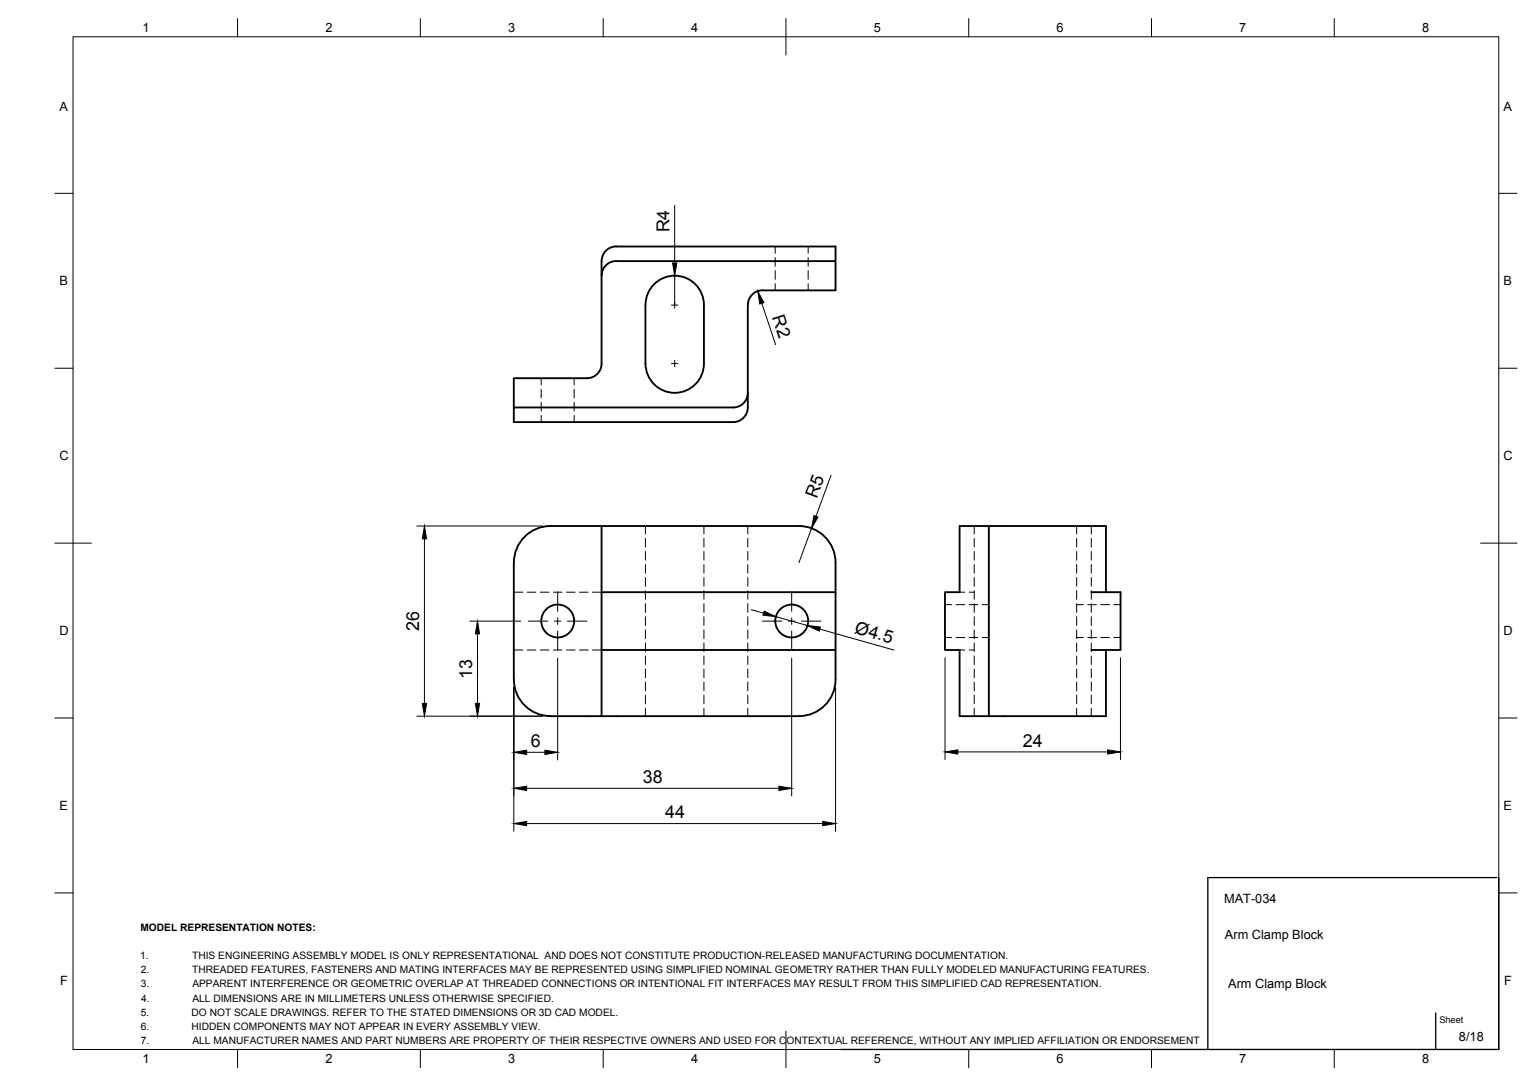
ISO-10303-21;
HEADER;
/* Generated by software containing ST-Developer
 * from STEP Tools, Inc. (www.steptools.com) 
 */

FILE_DESCRIPTION(
/* description */ ('STEP AP214'),
/* implementation_level */ '2;1');

FILE_NAME(
/* name */ 'Arm Clamp Block.step',
/* time_stamp */ '2026-11-14T09:24:36-08:00',
/* author */ (''),
/* organization */ (''),
/* preprocessor_version */ 'ST-DEVELOPER v20.2',
/* originating_system */ 'Autodesk Translation Framework v15.17.0.0',
/* authorisation */ '');

FILE_SCHEMA (('AUTOMOTIVE_DESIGN { 1 0 10303 214 3 1 1 }'));
ENDSEC;

DATA;
#10=MECHANICAL_DESIGN_GEOMETRIC_PRESENTATION_REPRESENTATION('',(#214),#18867);
#182=SHAPE_REPRESENTATION_RELATIONSHIP('SRR','None',#18946,#198);
#198=ADVANCED_BREP_SHAPE_REPRESENTATION('',(#238),#18862);
#214=STYLED_ITEM('',(#19026),#238);
#238=MANIFOLD_SOLID_BREP('Body1',#10969);
#356=FACE_BOUND('',#1900,.T.);
#357=FACE_BOUND('',#1905,.T.);
#358=FACE_BOUND('',#1908,.T.);
#359=FACE_BOUND('',#1910,.T.);
#360=FACE_BOUND('',#1924,.T.);
#361=FACE_BOUND('',#1928,.T.);
#666=PLANE('',#12022);
#667=PLANE('',#12024);
#668=PLANE('',#12026);
#669=PLANE('',#12028);
#670=PLANE('',#12029);
#671=PLANE('',#12032);
#672=PLANE('',#12033);
#673=PLANE('',#12035);
#674=PLANE('',#12036);
#675=PLANE('',#12039);
#676=PLANE('',#12040);
#677=PLANE('',#12047);
#678=PLANE('',#12055);
#679=PLANE('',#12057);
#680=PLANE('',#12064);
#681=PLANE('',#12067);
#682=PLANE('',#12070);
#683=PLANE('',#12071);
#684=PLANE('',#12074);
#685=PLANE('',#12077);
#1192=FACE_OUTER_BOUND('',#1893,.T.);
#1193=FACE_OUTER_BOUND('',#1894,.T.);
#1194=FACE_OUTER_BOUND('',#1895,.T.);
#1195=FACE_OUTER_BOUND('',#1896,.T.);
#1196=FACE_OUTER_BOUND('',#1897,.T.);
#1197=FACE_OUTER_BOUND('',#1898,.T.);
#1198=FACE_OUTER_BOUND('',#1899,.T.);
#1199=FACE_OUTER_BOUND('',#1901,.T.);
#1200=FACE_OUTER_BOUND('',#1902,.T.);
#1201=FACE_OUTER_BOUND('',#1903,.T.);
#1202=FACE_OUTER_BOUND('',#1904,.T.);
#1203=FACE_OUTER_BOUND('',#1906,.T.);
#1204=FACE_OUTER_BOUND('',#1907,.T.);
#1205=FACE_OUTER_BOUND('',#1909,.T.);
#1206=FACE_OUTER_BOUND('',#1911,.T.);
#1207=FACE_OUTER_BOUND('',#1912,.T.);
#1208=FACE_OUTER_BOUND('',#1913,.T.);
#1209=FACE_OUTER_BOUND('',#1914,.T.);
#1210=FACE_OUTER_BOUND('',#1915,.T.);
#1211=FACE_OUTER_BOUND('',#1916,.T.);
#1212=FACE_OUTER_BOUND('',#1917,.T.);
#1213=FACE_OUTER_BOUND('',#1918,.T.);
#1214=FACE_OUTER_BOUND('',#1919,.T.);
#1215=FACE_OUTER_BOUND('',#1920,.T.);
#1216=FACE_OUTER_BOUND('',#1921,.T.);
#1217=FACE_OUTER_BOUND('',#1922,.T.);
#1218=FACE_OUTER_BOUND('',#1923,.T.);
#1219=FACE_OUTER_BOUND('',#1925,.T.);
#1220=FACE_OUTER_BOUND('',#1926,.T.);
#1221=FACE_OUTER_BOUND('',#1927,.T.);
#1222=FACE_OUTER_BOUND('',#1929,.T.);
#1223=FACE_OUTER_BOUND('',#1930,.T.);
#1224=FACE_OUTER_BOUND('',#1931,.T.);
#1225=FACE_OUTER_BOUND('',#1932,.T.);
#1226=FACE_OUTER_BOUND('',#1933,.T.);
#1227=FACE_OUTER_BOUND('',#1934,.T.);
#1893=EDGE_LOOP('',(#9564,#9565,#9566,#9567));
#1894=EDGE_LOOP('',(#9568,#9569,#9570,#9571));
#1895=EDGE_LOOP('',(#9572,#9573,#9574,#9575,#9576));
#1896=EDGE_LOOP('',(#9577,#9578,#9579,#9580,#9581));
#1897=EDGE_LOOP('',(#9582,#9583,#9584,#9585,#9586));
#1898=EDGE_LOOP('',(#9587,#9588,#9589,#9590,#9591,#9592,#9593,#9594));
#1899=EDGE_LOOP('',(#9595,#9596,#9597,#9598,#9599,#9600));
#1900=EDGE_LOOP('',(#9601));
#1901=EDGE_LOOP('',(#9602,#9603,#9604,#9605,#9606,#9607,#9608,#9609));
#1902=EDGE_LOOP('',(#9610,#9611,#9612,#9613,#9614));
#1903=EDGE_LOOP('',(#9615,#9616,#9617,#9618,#9619,#9620,#9621,#9622));
#1904=EDGE_LOOP('',(#9623,#9624,#9625,#9626,#9627,#9628));
#1905=EDGE_LOOP('',(#9629));
#1906=EDGE_LOOP('',(#9630,#9631,#9632,#9633,#9634,#9635,#9636,#9637));
#1907=EDGE_LOOP('',(#9638,#9639,#9640,#9641,#9642,#9643,#9644,#9645,#9646,
#9647,#9648,#9649));
#1908=EDGE_LOOP('',(#9650,#9651,#9652,#9653));
#1909=EDGE_LOOP('',(#9654,#9655,#9656,#9657,#9658,#9659,#9660,#9661,#9662,
#9663,#9664,#9665));
#1910=EDGE_LOOP('',(#9666,#9667,#9668,#9669));
#1911=EDGE_LOOP('',(#9670,#9671,#9672,#9673));
#1912=EDGE_LOOP('',(#9674,#9675,#9676,#9677));
#1913=EDGE_LOOP('',(#9678,#9679,#9680,#9681));
#1914=EDGE_LOOP('',(#9682,#9683,#9684,#9685));
#1915=EDGE_LOOP('',(#9686,#9687,#9688,#9689));
#1916=EDGE_LOOP('',(#9690,#9691,#9692,#9693));
#1917=EDGE_LOOP('',(#9694,#9695,#9696,#9697));
#1918=EDGE_LOOP('',(#9698,#9699,#9700,#9701));
#1919=EDGE_LOOP('',(#9702,#9703,#9704,#9705));
#1920=EDGE_LOOP('',(#9706,#9707,#9708,#9709));
#1921=EDGE_LOOP('',(#9710,#9711,#9712,#9713,#9714,#9715));
#1922=EDGE_LOOP('',(#9716,#9717,#9718,#9719,#9720,#9721));
#1923=EDGE_LOOP('',(#9722,#9723,#9724,#9725));
#1924=EDGE_LOOP('',(#9726));
#1925=EDGE_LOOP('',(#9727,#9728,#9729,#9730,#9731,#9732));
#1926=EDGE_LOOP('',(#9733,#9734,#9735,#9736,#9737,#9738));
#1927=EDGE_LOOP('',(#9739,#9740,#9741,#9742));
#1928=EDGE_LOOP('',(#9743));
#1929=EDGE_LOOP('',(#9744,#9745,#9746,#9747));
#1930=EDGE_LOOP('',(#9748,#9749,#9750,#9751));
#1931=EDGE_LOOP('',(#9752,#9753,#9754,#9755));
#1932=EDGE_LOOP('',(#9756,#9757,#9758,#9759));
#1933=EDGE_LOOP('',(#9760,#9761,#9762,#9763));
#1934=EDGE_LOOP('',(#9764,#9765,#9766,#9767));
#2894=LINE('',#18183,#3908);
#2895=LINE('',#18189,#3909);
#2896=LINE('',#18194,#3910);
#2897=LINE('',#18196,#3911);
#2898=LINE('',#18198,#3912);
#2899=LINE('',#18200,#3913);
#2900=LINE('',#18205,#3914);
#2901=LINE('',#18207,#3915);
#2902=LINE('',#18209,#3916);
#2903=LINE('',#18211,#3917);
#2904=LINE('',#18216,#3918);
#2905=LINE('',#18218,#3919);
#2906=LINE('',#18220,#3920);
#2907=LINE('',#18223,#3921);
#2908=LINE('',#18226,#3922);
#2909=LINE('',#18228,#3923);
#2910=LINE('',#18229,#3924);
#2911=LINE('',#18231,#3925);
#2912=LINE('',#18233,#3926);
#2913=LINE('',#18234,#3927);
#2914=LINE('',#18239,#3928);
#2915=LINE('',#18241,#3929);
#2916=LINE('',#18243,#3930);
#2917=LINE('',#18248,#3931);
#2918=LINE('',#18250,#3932);
#2919=LINE('',#18252,#3933);
#2920=LINE('',#18254,#3934);
#2921=LINE('',#18256,#3935);
#2922=LINE('',#18258,#3936);
#2923=LINE('',#18260,#3937);
#2924=LINE('',#18261,#3938);
#2925=LINE('',#18265,#3939);
#2926=LINE('',#18267,#3940);
#2927=LINE('',#18269,#3941);
#2928=LINE('',#18272,#3942);
#2929=LINE('',#18276,#3943);
#2930=LINE('',#18277,#3944);
#2931=LINE('',#18279,#3945);
#2932=LINE('',#18281,#3946);
#2933=LINE('',#18282,#3947);
#2934=LINE('',#18283,#3948);
#2935=LINE('',#18287,#3949);
#2936=LINE('',#18292,#3950);
#2937=LINE('',#18293,#3951);
#2938=LINE('',#18297,#3952);
#2939=LINE('',#18299,#3953);
#2940=LINE('',#18301,#3954);
#2941=LINE('',#18303,#3955);
#2942=LINE('',#18305,#3956);
#2943=LINE('',#18307,#3957);
#2944=LINE('',#18309,#3958);
#2945=LINE('',#18310,#3959);
#2946=LINE('',#18313,#3960);
#2947=LINE('',#18316,#3961);
#2948=LINE('',#18322,#3962);
#2949=LINE('',#18325,#3963);
#2950=LINE('',#18329,#3964);
#2951=LINE('',#18332,#3965);
#2952=LINE('',#18335,#3966);
#2953=LINE('',#18339,#3967);
#2954=LINE('',#18342,#3968);
#2955=LINE('',#18343,#3969);
#2956=LINE('',#18345,#3970);
#2957=LINE('',#18347,#3971);
#2958=LINE('',#18359,#3972);
#2959=LINE('',#18362,#3973);
#2960=LINE('',#18366,#3974);
#2961=LINE('',#18371,#3975);
#2962=LINE('',#18374,#3976);
#2963=LINE('',#18378,#3977);
#3908=VECTOR('',#14868,2.25);
#3909=VECTOR('',#14875,2.25);
#3910=VECTOR('',#14880,1000.);
#3911=VECTOR('',#14881,1000.);
#3912=VECTOR('',#14882,1000.);
#3913=VECTOR('',#14883,1000.);
#3914=VECTOR('',#14888,1000.);
#3915=VECTOR('',#14889,1000.);
#3916=VECTOR('',#14890,1000.);
#3917=VECTOR('',#14891,1000.);
#3918=VECTOR('',#14896,1000.);
#3919=VECTOR('',#14897,1000.);
#3920=VECTOR('',#14898,1000.);
#3921=VECTOR('',#14901,1000.);
#3922=VECTOR('',#14904,1000.);
#3923=VECTOR('',#14905,1000.);
#3924=VECTOR('',#14906,1000.);
#3925=VECTOR('',#14907,1000.);
#3926=VECTOR('',#14908,1000.);
#3927=VECTOR('',#14909,1000.);
#3928=VECTOR('',#14914,1000.);
#3929=VECTOR('',#14915,1000.);
#3930=VECTOR('',#14916,1000.);
#3931=VECTOR('',#14921,1000.);
#3932=VECTOR('',#14922,1000.);
#3933=VECTOR('',#14923,1000.);
#3934=VECTOR('',#14924,1000.);
#3935=VECTOR('',#14925,1000.);
#3936=VECTOR('',#14926,1000.);
#3937=VECTOR('',#14927,1000.);
#3938=VECTOR('',#14928,1000.);
#3939=VECTOR('',#14931,1000.);
#3940=VECTOR('',#14932,1000.);
#3941=VECTOR('',#14933,1000.);
#3942=VECTOR('',#14936,1000.);
#3943=VECTOR('',#14939,1000.);
#3944=VECTOR('',#14940,1000.);
#3945=VECTOR('',#14941,1000.);
#3946=VECTOR('',#14942,1000.);
#3947=VECTOR('',#14943,1000.);
#3948=VECTOR('',#14944,1000.);
#3949=VECTOR('',#14947,1000.);
#3950=VECTOR('',#14952,1000.);
#3951=VECTOR('',#14953,1000.);
#3952=VECTOR('',#14956,1000.);
#3953=VECTOR('',#14957,1000.);
#3954=VECTOR('',#14958,1000.);
#3955=VECTOR('',#14959,1000.);
#3956=VECTOR('',#14960,1000.);
#3957=VECTOR('',#14961,1000.);
#3958=VECTOR('',#14962,1000.);
#3959=VECTOR('',#14963,1000.);
#3960=VECTOR('',#14968,1000.);
#3961=VECTOR('',#14973,1000.);
#3962=VECTOR('',#14978,1000.);
#3963=VECTOR('',#14981,1000.);
#3964=VECTOR('',#14988,1000.);
#3965=VECTOR('',#14993,1000.);
#3966=VECTOR('',#14994,1000.);
#3967=VECTOR('',#14997,1000.);
#3968=VECTOR('',#15002,1000.);
#3969=VECTOR('',#15003,1000.);
#3970=VECTOR('',#15006,1000.);
#3971=VECTOR('',#15009,1000.);
#3972=VECTOR('',#15030,1000.);
#3973=VECTOR('',#15033,1000.);
#3974=VECTOR('',#15040,1000.);
#3975=VECTOR('',#15047,1000.);
#3976=VECTOR('',#15050,1000.);
#3977=VECTOR('',#15057,1000.);
#4448=CIRCLE('',#12017,2.25);
#4449=CIRCLE('',#12018,2.25);
#4450=CIRCLE('',#12020,2.25);
#4451=CIRCLE('',#12021,2.25);
#4452=CIRCLE('',#12023,5.);
#4453=CIRCLE('',#12025,5.);
#4454=CIRCLE('',#12027,5.);
#4455=CIRCLE('',#12030,5.);
#4456=CIRCLE('',#12031,5.);
#4457=CIRCLE('',#12034,5.);
#4458=CIRCLE('',#12037,5.);
#4459=CIRCLE('',#12038,5.);
#4460=CIRCLE('',#12041,2.);
#4461=CIRCLE('',#12042,2.);
#4462=CIRCLE('',#12043,2.);
#4463=CIRCLE('',#12044,2.);
#4464=CIRCLE('',#12045,4.);
#4465=CIRCLE('',#12046,4.);
#4466=CIRCLE('',#12048,2.);
#4467=CIRCLE('',#12049,2.);
#4468=CIRCLE('',#12050,2.);
#4469=CIRCLE('',#12051,2.);
#4470=CIRCLE('',#12052,4.);
#4471=CIRCLE('',#12053,4.);
#4472=CIRCLE('',#12065,2.);
#4473=CIRCLE('',#12066,2.);
#4474=CIRCLE('',#12068,2.);
#4475=CIRCLE('',#12069,2.);
#4476=CIRCLE('',#12072,2.);
#4477=CIRCLE('',#12073,2.);
#4478=CIRCLE('',#12075,2.);
#4479=CIRCLE('',#12076,2.);
#5388=VERTEX_POINT('',#18180);
#5389=VERTEX_POINT('',#18182);
#5390=VERTEX_POINT('',#18186);
#5391=VERTEX_POINT('',#18188);
#5392=VERTEX_POINT('',#18192);
#5393=VERTEX_POINT('',#18193);
#5394=VERTEX_POINT('',#18195);
#5395=VERTEX_POINT('',#18197);
#5396=VERTEX_POINT('',#18199);
#5397=VERTEX_POINT('',#18203);
#5398=VERTEX_POINT('',#18204);
#5399=VERTEX_POINT('',#18206);
#5400=VERTEX_POINT('',#18208);
#5401=VERTEX_POINT('',#18210);
#5402=VERTEX_POINT('',#18214);
#5403=VERTEX_POINT('',#18215);
#5404=VERTEX_POINT('',#18217);
#5405=VERTEX_POINT('',#18219);
#5406=VERTEX_POINT('',#18221);
#5407=VERTEX_POINT('',#18225);
#5408=VERTEX_POINT('',#18227);
#5409=VERTEX_POINT('',#18230);
#5410=VERTEX_POINT('',#18232);
#5411=VERTEX_POINT('',#18236);
#5412=VERTEX_POINT('',#18238);
#5413=VERTEX_POINT('',#18240);
#5414=VERTEX_POINT('',#18242);
#5415=VERTEX_POINT('',#18246);
#5416=VERTEX_POINT('',#18247);
#5417=VERTEX_POINT('',#18249);
#5418=VERTEX_POINT('',#18251);
#5419=VERTEX_POINT('',#18253);
#5420=VERTEX_POINT('',#18255);
#5421=VERTEX_POINT('',#18257);
#5422=VERTEX_POINT('',#18259);
#5423=VERTEX_POINT('',#18263);
#5424=VERTEX_POINT('',#18264);
#5425=VERTEX_POINT('',#18266);
#5426=VERTEX_POINT('',#18268);
#5427=VERTEX_POINT('',#18270);
#5428=VERTEX_POINT('',#18274);
#5429=VERTEX_POINT('',#18275);
#5430=VERTEX_POINT('',#18278);
#5431=VERTEX_POINT('',#18280);
#5432=VERTEX_POINT('',#18285);
#5433=VERTEX_POINT('',#18286);
#5434=VERTEX_POINT('',#18289);
#5435=VERTEX_POINT('',#18291);
#5436=VERTEX_POINT('',#18295);
#5437=VERTEX_POINT('',#18296);
#5438=VERTEX_POINT('',#18298);
#5439=VERTEX_POINT('',#18300);
#5440=VERTEX_POINT('',#18302);
#5441=VERTEX_POINT('',#18304);
#5442=VERTEX_POINT('',#18306);
#5443=VERTEX_POINT('',#18308);
#5444=VERTEX_POINT('',#18318);
#5445=VERTEX_POINT('',#18319);
#5446=VERTEX_POINT('',#18321);
#5447=VERTEX_POINT('',#18323);
#5448=VERTEX_POINT('',#18333);
#5449=VERTEX_POINT('',#18334);
#5450=VERTEX_POINT('',#18336);
#5451=VERTEX_POINT('',#18338);
#5452=VERTEX_POINT('',#18357);
#5453=VERTEX_POINT('',#18361);
#5454=VERTEX_POINT('',#18369);
#5455=VERTEX_POINT('',#18373);
#6815=EDGE_CURVE('',#5388,#5388,#4448,.T.);
#6816=EDGE_CURVE('',#5388,#5389,#2894,.T.);
#6817=EDGE_CURVE('',#5389,#5389,#4449,.T.);
#6818=EDGE_CURVE('',#5390,#5390,#4450,.T.);
#6819=EDGE_CURVE('',#5390,#5391,#2895,.T.);
#6820=EDGE_CURVE('',#5391,#5391,#4451,.T.);
#6821=EDGE_CURVE('',#5392,#5393,#2896,.T.);
#6822=EDGE_CURVE('',#5392,#5394,#2897,.T.);
#6823=EDGE_CURVE('',#5395,#5394,#2898,.T.);
#6824=EDGE_CURVE('',#5396,#5395,#2899,.T.);
#6825=EDGE_CURVE('',#5396,#5393,#4452,.T.);
#6826=EDGE_CURVE('',#5397,#5398,#2900,.T.);
#6827=EDGE_CURVE('',#5398,#5399,#2901,.T.);
#6828=EDGE_CURVE('',#5399,#5400,#2902,.T.);
#6829=EDGE_CURVE('',#5401,#5400,#2903,.T.);
#6830=EDGE_CURVE('',#5401,#5397,#4453,.T.);
#6831=EDGE_CURVE('',#5402,#5403,#2904,.T.);
#6832=EDGE_CURVE('',#5402,#5404,#2905,.T.);
#6833=EDGE_CURVE('',#5405,#5404,#2906,.T.);
#6834=EDGE_CURVE('',#5405,#5406,#4454,.T.);
#6835=EDGE_CURVE('',#5403,#5406,#2907,.T.);
#6836=EDGE_CURVE('',#5407,#5400,#2908,.T.);
#6837=EDGE_CURVE('',#5408,#5407,#2909,.T.);
#6838=EDGE_CURVE('',#5408,#5403,#2910,.T.);
#6839=EDGE_CURVE('',#5406,#5409,#2911,.T.);
#6840=EDGE_CURVE('',#5410,#5409,#2912,.T.);
#6841=EDGE_CURVE('',#5410,#5401,#2913,.T.);
#6842=EDGE_CURVE('',#5409,#5411,#4455,.T.);
#6843=EDGE_CURVE('',#5412,#5411,#2914,.T.);
#6844=EDGE_CURVE('',#5412,#5413,#2915,.T.);
#6845=EDGE_CURVE('',#5413,#5414,#2916,.T.);
#6846=EDGE_CURVE('',#5414,#5410,#4456,.T.);
#6847=EDGE_CURVE('',#5415,#5416,#2917,.T.);
#6848=EDGE_CURVE('',#5415,#5417,#2918,.T.);
#6849=EDGE_CURVE('',#5417,#5418,#2919,.T.);
#6850=EDGE_CURVE('',#5418,#5419,#2920,.T.);
#6851=EDGE_CURVE('',#5419,#5420,#2921,.T.);
#6852=EDGE_CURVE('',#5420,#5421,#2922,.T.);
#6853=EDGE_CURVE('',#5421,#5422,#2923,.T.);
#6854=EDGE_CURVE('',#5422,#5416,#2924,.T.);
#6855=EDGE_CURVE('',#5423,#5424,#2925,.T.);
#6856=EDGE_CURVE('',#5424,#5425,#2926,.T.);
#6857=EDGE_CURVE('',#5425,#5426,#2927,.T.);
#6858=EDGE_CURVE('',#5426,#5427,#4457,.T.);
#6859=EDGE_CURVE('',#5423,#5427,#2928,.T.);
#6860=EDGE_CURVE('',#5428,#5429,#2929,.T.);
#6861=EDGE_CURVE('',#5428,#5396,#2930,.T.);
#6862=EDGE_CURVE('',#5430,#5395,#2931,.T.);
#6863=EDGE_CURVE('',#5431,#5430,#2932,.T.);
#6864=EDGE_CURVE('',#5431,#5423,#2933,.T.);
#6865=EDGE_CURVE('',#5427,#5429,#2934,.T.);
#6866=EDGE_CURVE('',#5432,#5433,#2935,.T.);
#6867=EDGE_CURVE('',#5433,#5428,#4458,.T.);
#6868=EDGE_CURVE('',#5429,#5434,#4459,.T.);
#6869=EDGE_CURVE('',#5435,#5434,#2936,.T.);
#6870=EDGE_CURVE('',#5435,#5432,#2937,.T.);
#6871=EDGE_CURVE('',#5436,#5437,#2938,.T.);
#6872=EDGE_CURVE('',#5437,#5438,#2939,.T.);
#6873=EDGE_CURVE('',#5438,#5439,#2940,.T.);
#6874=EDGE_CURVE('',#5439,#5440,#2941,.T.);
#6875=EDGE_CURVE('',#5440,#5441,#2942,.T.);
#6876=EDGE_CURVE('',#5441,#5442,#2943,.T.);
#6877=EDGE_CURVE('',#5443,#5442,#2944,.T.);
#6878=EDGE_CURVE('',#5443,#5436,#2945,.T.);
#6879=EDGE_CURVE('',#5442,#5398,#4460,.T.);
#6880=EDGE_CURVE('',#5397,#5414,#2946,.T.);
#6881=EDGE_CURVE('',#5413,#5422,#4461,.T.);
#6882=EDGE_CURVE('',#5421,#5392,#4462,.T.);
#6883=EDGE_CURVE('',#5393,#5433,#2947,.T.);
#6884=EDGE_CURVE('',#5432,#5443,#4463,.T.);
#6885=EDGE_CURVE('',#5444,#5445,#4464,.T.);
#6886=EDGE_CURVE('',#5446,#5444,#2948,.T.);
#6887=EDGE_CURVE('',#5447,#5446,#4465,.T.);
#6888=EDGE_CURVE('',#5445,#5447,#2949,.T.);
#6889=EDGE_CURVE('',#5404,#5437,#4466,.T.);
#6890=EDGE_CURVE('',#5436,#5435,#4467,.T.);
#6891=EDGE_CURVE('',#5434,#5426,#2950,.T.);
#6892=EDGE_CURVE('',#5425,#5415,#4468,.T.);
#6893=EDGE_CURVE('',#5416,#5412,#4469,.T.);
#6894=EDGE_CURVE('',#5411,#5405,#2951,.T.);
#6895=EDGE_CURVE('',#5448,#5449,#2952,.T.);
#6896=EDGE_CURVE('',#5449,#5450,#4470,.T.);
#6897=EDGE_CURVE('',#5450,#5451,#2953,.T.);
#6898=EDGE_CURVE('',#5451,#5448,#4471,.T.);
#6899=EDGE_CURVE('',#5450,#5445,#2954,.T.);
#6900=EDGE_CURVE('',#5449,#5444,#2955,.T.);
#6901=EDGE_CURVE('',#5448,#5446,#2956,.T.);
#6902=EDGE_CURVE('',#5451,#5447,#2957,.T.);
#6903=EDGE_CURVE('',#5399,#5441,#4472,.T.);
#6904=EDGE_CURVE('',#5440,#5452,#4473,.T.);
#6905=EDGE_CURVE('',#5452,#5407,#2958,.T.);
#6906=EDGE_CURVE('',#5453,#5408,#2959,.T.);
#6907=EDGE_CURVE('',#5453,#5439,#4474,.T.);
#6908=EDGE_CURVE('',#5438,#5402,#4475,.T.);
#6909=EDGE_CURVE('',#5452,#5453,#2960,.T.);
#6910=EDGE_CURVE('',#5394,#5420,#4476,.T.);
#6911=EDGE_CURVE('',#5419,#5454,#4477,.T.);
#6912=EDGE_CURVE('',#5430,#5454,#2961,.T.);
#6913=EDGE_CURVE('',#5431,#5455,#2962,.T.);
#6914=EDGE_CURVE('',#5455,#5418,#4478,.T.);
#6915=EDGE_CURVE('',#5417,#5424,#4479,.T.);
#6916=EDGE_CURVE('',#5454,#5455,#2963,.T.);
#9564=ORIENTED_EDGE('',*,*,#6815,.T.);
#9565=ORIENTED_EDGE('',*,*,#6816,.T.);
#9566=ORIENTED_EDGE('',*,*,#6817,.F.);
#9567=ORIENTED_EDGE('',*,*,#6816,.F.);
#9568=ORIENTED_EDGE('',*,*,#6818,.F.);
#9569=ORIENTED_EDGE('',*,*,#6819,.T.);
#9570=ORIENTED_EDGE('',*,*,#6820,.T.);
#9571=ORIENTED_EDGE('',*,*,#6819,.F.);
#9572=ORIENTED_EDGE('',*,*,#6821,.F.);
#9573=ORIENTED_EDGE('',*,*,#6822,.T.);
#9574=ORIENTED_EDGE('',*,*,#6823,.F.);
#9575=ORIENTED_EDGE('',*,*,#6824,.F.);
#9576=ORIENTED_EDGE('',*,*,#6825,.T.);
#9577=ORIENTED_EDGE('',*,*,#6826,.T.);
#9578=ORIENTED_EDGE('',*,*,#6827,.T.);
#9579=ORIENTED_EDGE('',*,*,#6828,.T.);
#9580=ORIENTED_EDGE('',*,*,#6829,.F.);
#9581=ORIENTED_EDGE('',*,*,#6830,.T.);
#9582=ORIENTED_EDGE('',*,*,#6831,.F.);
#9583=ORIENTED_EDGE('',*,*,#6832,.T.);
#9584=ORIENTED_EDGE('',*,*,#6833,.F.);
#9585=ORIENTED_EDGE('',*,*,#6834,.T.);
#9586=ORIENTED_EDGE('',*,*,#6835,.F.);
#9587=ORIENTED_EDGE('',*,*,#6829,.T.);
#9588=ORIENTED_EDGE('',*,*,#6836,.F.);
#9589=ORIENTED_EDGE('',*,*,#6837,.F.);
#9590=ORIENTED_EDGE('',*,*,#6838,.T.);
#9591=ORIENTED_EDGE('',*,*,#6835,.T.);
#9592=ORIENTED_EDGE('',*,*,#6839,.T.);
#9593=ORIENTED_EDGE('',*,*,#6840,.F.);
#9594=ORIENTED_EDGE('',*,*,#6841,.T.);
#9595=ORIENTED_EDGE('',*,*,#6840,.T.);
#9596=ORIENTED_EDGE('',*,*,#6842,.T.);
#9597=ORIENTED_EDGE('',*,*,#6843,.F.);
#9598=ORIENTED_EDGE('',*,*,#6844,.T.);
#9599=ORIENTED_EDGE('',*,*,#6845,.T.);
#9600=ORIENTED_EDGE('',*,*,#6846,.T.);
#9601=ORIENTED_EDGE('',*,*,#6815,.F.);
#9602=ORIENTED_EDGE('',*,*,#6847,.F.);
#9603=ORIENTED_EDGE('',*,*,#6848,.T.);
#9604=ORIENTED_EDGE('',*,*,#6849,.T.);
#9605=ORIENTED_EDGE('',*,*,#6850,.T.);
#9606=ORIENTED_EDGE('',*,*,#6851,.T.);
#9607=ORIENTED_EDGE('',*,*,#6852,.T.);
#9608=ORIENTED_EDGE('',*,*,#6853,.T.);
#9609=ORIENTED_EDGE('',*,*,#6854,.T.);
#9610=ORIENTED_EDGE('',*,*,#6855,.T.);
#9611=ORIENTED_EDGE('',*,*,#6856,.T.);
#9612=ORIENTED_EDGE('',*,*,#6857,.T.);
#9613=ORIENTED_EDGE('',*,*,#6858,.T.);
#9614=ORIENTED_EDGE('',*,*,#6859,.F.);
#9615=ORIENTED_EDGE('',*,*,#6860,.F.);
#9616=ORIENTED_EDGE('',*,*,#6861,.T.);
#9617=ORIENTED_EDGE('',*,*,#6824,.T.);
#9618=ORIENTED_EDGE('',*,*,#6862,.F.);
#9619=ORIENTED_EDGE('',*,*,#6863,.F.);
#9620=ORIENTED_EDGE('',*,*,#6864,.T.);
#9621=ORIENTED_EDGE('',*,*,#6859,.T.);
#9622=ORIENTED_EDGE('',*,*,#6865,.T.);
#9623=ORIENTED_EDGE('',*,*,#6866,.T.);
#9624=ORIENTED_EDGE('',*,*,#6867,.T.);
#9625=ORIENTED_EDGE('',*,*,#6860,.T.);
#9626=ORIENTED_EDGE('',*,*,#6868,.T.);
#9627=ORIENTED_EDGE('',*,*,#6869,.F.);
#9628=ORIENTED_EDGE('',*,*,#6870,.T.);
#9629=ORIENTED_EDGE('',*,*,#6820,.F.);
#9630=ORIENTED_EDGE('',*,*,#6871,.T.);
#9631=ORIENTED_EDGE('',*,*,#6872,.T.);
#9632=ORIENTED_EDGE('',*,*,#6873,.T.);
#9633=ORIENTED_EDGE('',*,*,#6874,.T.);
#9634=ORIENTED_EDGE('',*,*,#6875,.T.);
#9635=ORIENTED_EDGE('',*,*,#6876,.T.);
#9636=ORIENTED_EDGE('',*,*,#6877,.F.);
#9637=ORIENTED_EDGE('',*,*,#6878,.T.);
#9638=ORIENTED_EDGE('',*,*,#6877,.T.);
#9639=ORIENTED_EDGE('',*,*,#6879,.T.);
#9640=ORIENTED_EDGE('',*,*,#6826,.F.);
#9641=ORIENTED_EDGE('',*,*,#6880,.T.);
#9642=ORIENTED_EDGE('',*,*,#6845,.F.);
#9643=ORIENTED_EDGE('',*,*,#6881,.T.);
#9644=ORIENTED_EDGE('',*,*,#6853,.F.);
#9645=ORIENTED_EDGE('',*,*,#6882,.T.);
#9646=ORIENTED_EDGE('',*,*,#6821,.T.);
#9647=ORIENTED_EDGE('',*,*,#6883,.T.);
#9648=ORIENTED_EDGE('',*,*,#6866,.F.);
#9649=ORIENTED_EDGE('',*,*,#6884,.T.);
#9650=ORIENTED_EDGE('',*,*,#6885,.F.);
#9651=ORIENTED_EDGE('',*,*,#6886,.F.);
#9652=ORIENTED_EDGE('',*,*,#6887,.F.);
#9653=ORIENTED_EDGE('',*,*,#6888,.F.);
#9654=ORIENTED_EDGE('',*,*,#6833,.T.);
#9655=ORIENTED_EDGE('',*,*,#6889,.T.);
#9656=ORIENTED_EDGE('',*,*,#6871,.F.);
#9657=ORIENTED_EDGE('',*,*,#6890,.T.);
#9658=ORIENTED_EDGE('',*,*,#6869,.T.);
#9659=ORIENTED_EDGE('',*,*,#6891,.T.);
#9660=ORIENTED_EDGE('',*,*,#6857,.F.);
#9661=ORIENTED_EDGE('',*,*,#6892,.T.);
#9662=ORIENTED_EDGE('',*,*,#6847,.T.);
#9663=ORIENTED_EDGE('',*,*,#6893,.T.);
#9664=ORIENTED_EDGE('',*,*,#6843,.T.);
#9665=ORIENTED_EDGE('',*,*,#6894,.T.);
#9666=ORIENTED_EDGE('',*,*,#6895,.T.);
#9667=ORIENTED_EDGE('',*,*,#6896,.T.);
#9668=ORIENTED_EDGE('',*,*,#6897,.T.);
#9669=ORIENTED_EDGE('',*,*,#6898,.T.);
#9670=ORIENTED_EDGE('',*,*,#6885,.T.);
#9671=ORIENTED_EDGE('',*,*,#6899,.F.);
#9672=ORIENTED_EDGE('',*,*,#6896,.F.);
#9673=ORIENTED_EDGE('',*,*,#6900,.T.);
#9674=ORIENTED_EDGE('',*,*,#6886,.T.);
#9675=ORIENTED_EDGE('',*,*,#6900,.F.);
#9676=ORIENTED_EDGE('',*,*,#6895,.F.);
#9677=ORIENTED_EDGE('',*,*,#6901,.T.);
#9678=ORIENTED_EDGE('',*,*,#6887,.T.);
#9679=ORIENTED_EDGE('',*,*,#6901,.F.);
#9680=ORIENTED_EDGE('',*,*,#6898,.F.);
#9681=ORIENTED_EDGE('',*,*,#6902,.T.);
#9682=ORIENTED_EDGE('',*,*,#6888,.T.);
#9683=ORIENTED_EDGE('',*,*,#6902,.F.);
#9684=ORIENTED_EDGE('',*,*,#6897,.F.);
#9685=ORIENTED_EDGE('',*,*,#6899,.T.);
#9686=ORIENTED_EDGE('',*,*,#6884,.F.);
#9687=ORIENTED_EDGE('',*,*,#6870,.F.);
#9688=ORIENTED_EDGE('',*,*,#6890,.F.);
#9689=ORIENTED_EDGE('',*,*,#6878,.F.);
#9690=ORIENTED_EDGE('',*,*,#6881,.F.);
#9691=ORIENTED_EDGE('',*,*,#6844,.F.);
#9692=ORIENTED_EDGE('',*,*,#6893,.F.);
#9693=ORIENTED_EDGE('',*,*,#6854,.F.);
#9694=ORIENTED_EDGE('',*,*,#6825,.F.);
#9695=ORIENTED_EDGE('',*,*,#6861,.F.);
#9696=ORIENTED_EDGE('',*,*,#6867,.F.);
#9697=ORIENTED_EDGE('',*,*,#6883,.F.);
#9698=ORIENTED_EDGE('',*,*,#6858,.F.);
#9699=ORIENTED_EDGE('',*,*,#6891,.F.);
#9700=ORIENTED_EDGE('',*,*,#6868,.F.);
#9701=ORIENTED_EDGE('',*,*,#6865,.F.);
#9702=ORIENTED_EDGE('',*,*,#6834,.F.);
#9703=ORIENTED_EDGE('',*,*,#6894,.F.);
#9704=ORIENTED_EDGE('',*,*,#6842,.F.);
#9705=ORIENTED_EDGE('',*,*,#6839,.F.);
#9706=ORIENTED_EDGE('',*,*,#6830,.F.);
#9707=ORIENTED_EDGE('',*,*,#6841,.F.);
#9708=ORIENTED_EDGE('',*,*,#6846,.F.);
#9709=ORIENTED_EDGE('',*,*,#6880,.F.);
#9710=ORIENTED_EDGE('',*,*,#6828,.F.);
#9711=ORIENTED_EDGE('',*,*,#6903,.T.);
#9712=ORIENTED_EDGE('',*,*,#6875,.F.);
#9713=ORIENTED_EDGE('',*,*,#6904,.T.);
#9714=ORIENTED_EDGE('',*,*,#6905,.T.);
#9715=ORIENTED_EDGE('',*,*,#6836,.T.);
#9716=ORIENTED_EDGE('',*,*,#6906,.F.);
#9717=ORIENTED_EDGE('',*,*,#6907,.T.);
#9718=ORIENTED_EDGE('',*,*,#6873,.F.);
#9719=ORIENTED_EDGE('',*,*,#6908,.T.);
#9720=ORIENTED_EDGE('',*,*,#6831,.T.);
#9721=ORIENTED_EDGE('',*,*,#6838,.F.);
#9722=ORIENTED_EDGE('',*,*,#6905,.F.);
#9723=ORIENTED_EDGE('',*,*,#6909,.T.);
#9724=ORIENTED_EDGE('',*,*,#6906,.T.);
#9725=ORIENTED_EDGE('',*,*,#6837,.T.);
#9726=ORIENTED_EDGE('',*,*,#6817,.T.);
#9727=ORIENTED_EDGE('',*,*,#6823,.T.);
#9728=ORIENTED_EDGE('',*,*,#6910,.T.);
#9729=ORIENTED_EDGE('',*,*,#6851,.F.);
#9730=ORIENTED_EDGE('',*,*,#6911,.T.);
#9731=ORIENTED_EDGE('',*,*,#6912,.F.);
#9732=ORIENTED_EDGE('',*,*,#6862,.T.);
#9733=ORIENTED_EDGE('',*,*,#6913,.T.);
#9734=ORIENTED_EDGE('',*,*,#6914,.T.);
#9735=ORIENTED_EDGE('',*,*,#6849,.F.);
#9736=ORIENTED_EDGE('',*,*,#6915,.T.);
#9737=ORIENTED_EDGE('',*,*,#6855,.F.);
#9738=ORIENTED_EDGE('',*,*,#6864,.F.);
#9739=ORIENTED_EDGE('',*,*,#6912,.T.);
#9740=ORIENTED_EDGE('',*,*,#6916,.T.);
#9741=ORIENTED_EDGE('',*,*,#6913,.F.);
#9742=ORIENTED_EDGE('',*,*,#6863,.T.);
#9743=ORIENTED_EDGE('',*,*,#6818,.T.);
#9744=ORIENTED_EDGE('',*,*,#6889,.F.);
#9745=ORIENTED_EDGE('',*,*,#6832,.F.);
#9746=ORIENTED_EDGE('',*,*,#6908,.F.);
#9747=ORIENTED_EDGE('',*,*,#6872,.F.);
#9748=ORIENTED_EDGE('',*,*,#6907,.F.);
#9749=ORIENTED_EDGE('',*,*,#6909,.F.);
#9750=ORIENTED_EDGE('',*,*,#6904,.F.);
#9751=ORIENTED_EDGE('',*,*,#6874,.F.);
#9752=ORIENTED_EDGE('',*,*,#6903,.F.);
#9753=ORIENTED_EDGE('',*,*,#6827,.F.);
#9754=ORIENTED_EDGE('',*,*,#6879,.F.);
#9755=ORIENTED_EDGE('',*,*,#6876,.F.);
#9756=ORIENTED_EDGE('',*,*,#6915,.F.);
#9757=ORIENTED_EDGE('',*,*,#6848,.F.);
#9758=ORIENTED_EDGE('',*,*,#6892,.F.);
#9759=ORIENTED_EDGE('',*,*,#6856,.F.);
#9760=ORIENTED_EDGE('',*,*,#6914,.F.);
#9761=ORIENTED_EDGE('',*,*,#6916,.F.);
#9762=ORIENTED_EDGE('',*,*,#6911,.F.);
#9763=ORIENTED_EDGE('',*,*,#6850,.F.);
#9764=ORIENTED_EDGE('',*,*,#6882,.F.);
#9765=ORIENTED_EDGE('',*,*,#6852,.F.);
#9766=ORIENTED_EDGE('',*,*,#6910,.F.);
#9767=ORIENTED_EDGE('',*,*,#6822,.F.);
#10321=CYLINDRICAL_SURFACE('',#12016,2.25);
#10322=CYLINDRICAL_SURFACE('',#12019,2.25);
#10323=CYLINDRICAL_SURFACE('',#12054,4.);
#10324=CYLINDRICAL_SURFACE('',#12056,4.);
#10325=CYLINDRICAL_SURFACE('',#12058,2.);
#10326=CYLINDRICAL_SURFACE('',#12059,2.);
#10327=CYLINDRICAL_SURFACE('',#12060,5.);
#10328=CYLINDRICAL_SURFACE('',#12061,5.);
#10329=CYLINDRICAL_SURFACE('',#12062,5.);
#10330=CYLINDRICAL_SURFACE('',#12063,5.);
#10331=CYLINDRICAL_SURFACE('',#12078,2.);
#10332=CYLINDRICAL_SURFACE('',#12079,2.);
#10333=CYLINDRICAL_SURFACE('',#12080,2.);
#10334=CYLINDRICAL_SURFACE('',#12081,2.);
#10335=CYLINDRICAL_SURFACE('',#12082,2.);
#10336=CYLINDRICAL_SURFACE('',#12083,2.);
#10829=ADVANCED_FACE('',(#1192),#10321,.F.);
#10830=ADVANCED_FACE('',(#1193),#10322,.F.);
#10831=ADVANCED_FACE('',(#1194),#666,.F.);
#10832=ADVANCED_FACE('',(#1195),#667,.T.);
#10833=ADVANCED_FACE('',(#1196),#668,.T.);
#10834=ADVANCED_FACE('',(#1197),#669,.F.);
#10835=ADVANCED_FACE('',(#1198,#356),#670,.T.);
#10836=ADVANCED_FACE('',(#1199),#671,.T.);
#10837=ADVANCED_FACE('',(#1200),#672,.F.);
#10838=ADVANCED_FACE('',(#1201),#673,.F.);
#10839=ADVANCED_FACE('',(#1202,#357),#674,.T.);
#10840=ADVANCED_FACE('',(#1203),#675,.F.);
#10841=ADVANCED_FACE('',(#1204,#358),#676,.T.);
#10842=ADVANCED_FACE('',(#1205,#359),#677,.F.);
#10843=ADVANCED_FACE('',(#1206),#10323,.F.);
#10844=ADVANCED_FACE('',(#1207),#678,.F.);
#10845=ADVANCED_FACE('',(#1208),#10324,.F.);
#10846=ADVANCED_FACE('',(#1209),#679,.F.);
#10847=ADVANCED_FACE('',(#1210),#10325,.F.);
#10848=ADVANCED_FACE('',(#1211),#10326,.F.);
#10849=ADVANCED_FACE('',(#1212),#10327,.T.);
#10850=ADVANCED_FACE('',(#1213),#10328,.T.);
#10851=ADVANCED_FACE('',(#1214),#10329,.T.);
#10852=ADVANCED_FACE('',(#1215),#10330,.T.);
#10853=ADVANCED_FACE('',(#1216),#680,.T.);
#10854=ADVANCED_FACE('',(#1217),#681,.F.);
#10855=ADVANCED_FACE('',(#1218,#360),#682,.T.);
#10856=ADVANCED_FACE('',(#1219),#683,.F.);
#10857=ADVANCED_FACE('',(#1220),#684,.T.);
#10858=ADVANCED_FACE('',(#1221,#361),#685,.T.);
#10859=ADVANCED_FACE('',(#1222),#10331,.T.);
#10860=ADVANCED_FACE('',(#1223),#10332,.T.);
#10861=ADVANCED_FACE('',(#1224),#10333,.T.);
#10862=ADVANCED_FACE('',(#1225),#10334,.T.);
#10863=ADVANCED_FACE('',(#1226),#10335,.T.);
#10864=ADVANCED_FACE('',(#1227),#10336,.T.);
#10969=CLOSED_SHELL('',(#10829,#10830,#10831,#10832,#10833,#10834,#10835,
#10836,#10837,#10838,#10839,#10840,#10841,#10842,#10843,#10844,#10845,#10846,
#10847,#10848,#10849,#10850,#10851,#10852,#10853,#10854,#10855,#10856,#10857,
#10858,#10859,#10860,#10861,#10862,#10863,#10864));
#12015=AXIS2_PLACEMENT_3D('',#18178,#14862,#14863);
#12016=AXIS2_PLACEMENT_3D('',#18179,#14864,#14865);
#12017=AXIS2_PLACEMENT_3D('',#18181,#14866,#14867);
#12018=AXIS2_PLACEMENT_3D('',#18184,#14869,#14870);
#12019=AXIS2_PLACEMENT_3D('',#18185,#14871,#14872);
#12020=AXIS2_PLACEMENT_3D('',#18187,#14873,#14874);
#12021=AXIS2_PLACEMENT_3D('',#18190,#14876,#14877);
#12022=AXIS2_PLACEMENT_3D('',#18191,#14878,#14879);
#12023=AXIS2_PLACEMENT_3D('',#18201,#14884,#14885);
#12024=AXIS2_PLACEMENT_3D('',#18202,#14886,#14887);
#12025=AXIS2_PLACEMENT_3D('',#18212,#14892,#14893);
#12026=AXIS2_PLACEMENT_3D('',#18213,#14894,#14895);
#12027=AXIS2_PLACEMENT_3D('',#18222,#14899,#14900);
#12028=AXIS2_PLACEMENT_3D('',#18224,#14902,#14903);
#12029=AXIS2_PLACEMENT_3D('',#18235,#14910,#14911);
#12030=AXIS2_PLACEMENT_3D('',#18237,#14912,#14913);
#12031=AXIS2_PLACEMENT_3D('',#18244,#14917,#14918);
#12032=AXIS2_PLACEMENT_3D('',#18245,#14919,#14920);
#12033=AXIS2_PLACEMENT_3D('',#18262,#14929,#14930);
#12034=AXIS2_PLACEMENT_3D('',#18271,#14934,#14935);
#12035=AXIS2_PLACEMENT_3D('',#18273,#14937,#14938);
#12036=AXIS2_PLACEMENT_3D('',#18284,#14945,#14946);
#12037=AXIS2_PLACEMENT_3D('',#18288,#14948,#14949);
#12038=AXIS2_PLACEMENT_3D('',#18290,#14950,#14951);
#12039=AXIS2_PLACEMENT_3D('',#18294,#14954,#14955);
#12040=AXIS2_PLACEMENT_3D('',#18311,#14964,#14965);
#12041=AXIS2_PLACEMENT_3D('',#18312,#14966,#14967);
#12042=AXIS2_PLACEMENT_3D('',#18314,#14969,#14970);
#12043=AXIS2_PLACEMENT_3D('',#18315,#14971,#14972);
#12044=AXIS2_PLACEMENT_3D('',#18317,#14974,#14975);
#12045=AXIS2_PLACEMENT_3D('',#18320,#14976,#14977);
#12046=AXIS2_PLACEMENT_3D('',#18324,#14979,#14980);
#12047=AXIS2_PLACEMENT_3D('',#18326,#14982,#14983);
#12048=AXIS2_PLACEMENT_3D('',#18327,#14984,#14985);
#12049=AXIS2_PLACEMENT_3D('',#18328,#14986,#14987);
#12050=AXIS2_PLACEMENT_3D('',#18330,#14989,#14990);
#12051=AXIS2_PLACEMENT_3D('',#18331,#14991,#14992);
#12052=AXIS2_PLACEMENT_3D('',#18337,#14995,#14996);
#12053=AXIS2_PLACEMENT_3D('',#18340,#14998,#14999);
#12054=AXIS2_PLACEMENT_3D('',#18341,#15000,#15001);
#12055=AXIS2_PLACEMENT_3D('',#18344,#15004,#15005);
#12056=AXIS2_PLACEMENT_3D('',#18346,#15007,#15008);
#12057=AXIS2_PLACEMENT_3D('',#18348,#15010,#15011);
#12058=AXIS2_PLACEMENT_3D('',#18349,#15012,#15013);
#12059=AXIS2_PLACEMENT_3D('',#18350,#15014,#15015);
#12060=AXIS2_PLACEMENT_3D('',#18351,#15016,#15017);
#12061=AXIS2_PLACEMENT_3D('',#18352,#15018,#15019);
#12062=AXIS2_PLACEMENT_3D('',#18353,#15020,#15021);
#12063=AXIS2_PLACEMENT_3D('',#18354,#15022,#15023);
#12064=AXIS2_PLACEMENT_3D('',#18355,#15024,#15025);
#12065=AXIS2_PLACEMENT_3D('',#18356,#15026,#15027);
#12066=AXIS2_PLACEMENT_3D('',#18358,#15028,#15029);
#12067=AXIS2_PLACEMENT_3D('',#18360,#15031,#15032);
#12068=AXIS2_PLACEMENT_3D('',#18363,#15034,#15035);
#12069=AXIS2_PLACEMENT_3D('',#18364,#15036,#15037);
#12070=AXIS2_PLACEMENT_3D('',#18365,#15038,#15039);
#12071=AXIS2_PLACEMENT_3D('',#18367,#15041,#15042);
#12072=AXIS2_PLACEMENT_3D('',#18368,#15043,#15044);
#12073=AXIS2_PLACEMENT_3D('',#18370,#15045,#15046);
#12074=AXIS2_PLACEMENT_3D('',#18372,#15048,#15049);
#12075=AXIS2_PLACEMENT_3D('',#18375,#15051,#15052);
#12076=AXIS2_PLACEMENT_3D('',#18376,#15053,#15054);
#12077=AXIS2_PLACEMENT_3D('',#18377,#15055,#15056);
#12078=AXIS2_PLACEMENT_3D('',#18379,#15058,#15059);
#12079=AXIS2_PLACEMENT_3D('',#18380,#15060,#15061);
#12080=AXIS2_PLACEMENT_3D('',#18381,#15062,#15063);
#12081=AXIS2_PLACEMENT_3D('',#18382,#15064,#15065);
#12082=AXIS2_PLACEMENT_3D('',#18383,#15066,#15067);
#12083=AXIS2_PLACEMENT_3D('',#18384,#15068,#15069);
#14862=DIRECTION('axis',(0.,0.,1.));
#14863=DIRECTION('refdir',(1.,0.,0.));
#14864=DIRECTION('center_axis',(-1.,0.,0.));
#14865=DIRECTION('ref_axis',(0.,0.,1.));
#14866=DIRECTION('center_axis',(1.,0.,4.33680868994202E-16));
#14867=DIRECTION('ref_axis',(4.33680868994202E-16,0.,-1.));
#14868=DIRECTION('',(-1.,0.,0.));
#14869=DIRECTION('center_axis',(1.,0.,0.));
#14870=DIRECTION('ref_axis',(0.,0.,1.));
#14871=DIRECTION('center_axis',(-1.,0.,0.));
#14872=DIRECTION('ref_axis',(0.,0.,1.));
#14873=DIRECTION('center_axis',(-1.,0.,0.));
#14874=DIRECTION('ref_axis',(0.,0.,-1.));
#14875=DIRECTION('',(-1.,0.,0.));
#14876=DIRECTION('center_axis',(-1.,0.,0.));
#14877=DIRECTION('ref_axis',(0.,0.,1.));
#14878=DIRECTION('center_axis',(-1.,0.,0.));
#14879=DIRECTION('ref_axis',(0.,0.,1.));
#14880=DIRECTION('',(0.,0.,-1.));
#14881=DIRECTION('',(0.,-1.,0.));
#14882=DIRECTION('',(0.,0.,1.));
#14883=DIRECTION('',(0.,-1.,0.));
#14884=DIRECTION('center_axis',(1.,0.,0.));
#14885=DIRECTION('ref_axis',(0.,0.,1.));
#14886=DIRECTION('center_axis',(-1.,0.,0.));
#14887=DIRECTION('ref_axis',(0.,0.,1.));
#14888=DIRECTION('',(0.,0.,-1.));
#14889=DIRECTION('',(0.,-1.,0.));
#14890=DIRECTION('',(0.,0.,1.));
#14891=DIRECTION('',(0.,-1.,0.));
#14892=DIRECTION('center_axis',(-1.,0.,0.));
#14893=DIRECTION('ref_axis',(0.,0.,1.));
#14894=DIRECTION('center_axis',(-1.,0.,0.));
#14895=DIRECTION('ref_axis',(0.,0.,1.));
#14896=DIRECTION('',(0.,0.,1.));
#14897=DIRECTION('',(0.,-1.,0.));
#14898=DIRECTION('',(0.,0.,-1.));
#14899=DIRECTION('center_axis',(-1.,0.,0.));
#14900=DIRECTION('ref_axis',(0.,0.,1.));
#14901=DIRECTION('',(0.,-1.,0.));
#14902=DIRECTION('center_axis',(0.,0.,-1.));
#14903=DIRECTION('ref_axis',(-1.,0.,0.));
#14904=DIRECTION('',(1.,0.,0.));
#14905=DIRECTION('',(0.,1.,0.));
#14906=DIRECTION('',(1.,0.,0.));
#14907=DIRECTION('',(1.,0.,0.));
#14908=DIRECTION('',(0.,-1.,0.));
#14909=DIRECTION('',(-1.,0.,0.));
#14910=DIRECTION('center_axis',(1.,0.,4.33680868994202E-16));
#14911=DIRECTION('ref_axis',(4.33680868994202E-16,0.,-1.));
#14912=DIRECTION('center_axis',(1.,0.,4.33680868994202E-16));
#14913=DIRECTION('ref_axis',(4.33680868994202E-16,0.,-1.));
#14914=DIRECTION('',(-4.33680868994202E-16,0.,1.));
#14915=DIRECTION('',(0.,1.,0.));
#14916=DIRECTION('',(-4.33680868994202E-16,0.,1.));
#14917=DIRECTION('center_axis',(1.,0.,4.33680868994202E-16));
#14918=DIRECTION('ref_axis',(4.33680868994202E-16,0.,-1.));
#14919=DIRECTION('center_axis',(1.73472347597681E-16,0.,1.));
#14920=DIRECTION('ref_axis',(1.,0.,-1.73472347597681E-16));
#14921=DIRECTION('',(-1.,0.,1.73472347597681E-16));
#14922=DIRECTION('',(0.,1.,0.));
#14923=DIRECTION('',(1.,0.,0.));
#14924=DIRECTION('',(0.,1.,0.));
#14925=DIRECTION('',(-1.,0.,0.));
#14926=DIRECTION('',(0.,1.,0.));
#14927=DIRECTION('',(-1.,0.,1.73472347597681E-16));
#14928=DIRECTION('',(0.,-1.,0.));
#14929=DIRECTION('center_axis',(-1.,0.,0.));
#14930=DIRECTION('ref_axis',(0.,0.,1.));
#14931=DIRECTION('',(0.,0.,1.));
#14932=DIRECTION('',(0.,-1.,0.));
#14933=DIRECTION('',(0.,0.,-1.));
#14934=DIRECTION('center_axis',(1.,0.,0.));
#14935=DIRECTION('ref_axis',(0.,0.,1.));
#14936=DIRECTION('',(0.,-1.,0.));
#14937=DIRECTION('center_axis',(0.,0.,1.));
#14938=DIRECTION('ref_axis',(1.,0.,0.));
#14939=DIRECTION('',(0.,-1.,0.));
#14940=DIRECTION('',(1.,0.,0.));
#14941=DIRECTION('',(-1.,0.,0.));
#14942=DIRECTION('',(0.,1.,0.));
#14943=DIRECTION('',(-1.,0.,0.));
#14944=DIRECTION('',(-1.,0.,0.));
#14945=DIRECTION('center_axis',(-1.,0.,0.));
#14946=DIRECTION('ref_axis',(0.,0.,1.));
#14947=DIRECTION('',(0.,0.,-1.));
#14948=DIRECTION('center_axis',(-1.,0.,0.));
#14949=DIRECTION('ref_axis',(0.,0.,1.));
#14950=DIRECTION('center_axis',(-1.,0.,0.));
#14951=DIRECTION('ref_axis',(0.,0.,1.));
#14952=DIRECTION('',(0.,0.,-1.));
#14953=DIRECTION('',(0.,1.,0.));
#14954=DIRECTION('center_axis',(0.,0.,1.));
#14955=DIRECTION('ref_axis',(1.,0.,0.));
#14956=DIRECTION('',(-1.,0.,0.));
#14957=DIRECTION('',(0.,1.,0.));
#14958=DIRECTION('',(-1.,0.,-7.2280144832367E-17));
#14959=DIRECTION('',(0.,1.,0.));
#14960=DIRECTION('',(1.,0.,7.2280144832367E-17));
#14961=DIRECTION('',(0.,1.,0.));
#14962=DIRECTION('',(-1.,0.,0.));
#14963=DIRECTION('',(0.,-1.,0.));
#14964=DIRECTION('center_axis',(0.,1.,0.));
#14965=DIRECTION('ref_axis',(0.,0.,1.));
#14966=DIRECTION('center_axis',(0.,1.,0.));
#14967=DIRECTION('ref_axis',(0.,0.,1.));
#14968=DIRECTION('',(1.,0.,0.));
#14969=DIRECTION('center_axis',(0.,-1.,0.));
#14970=DIRECTION('ref_axis',(0.,0.,1.));
#14971=DIRECTION('center_axis',(0.,1.,0.));
#14972=DIRECTION('ref_axis',(0.,0.,1.));
#14973=DIRECTION('',(-1.,0.,0.));
#14974=DIRECTION('center_axis',(0.,-1.,0.));
#14975=DIRECTION('ref_axis',(0.,0.,1.));
#14976=DIRECTION('center_axis',(0.,1.,0.));
#14977=DIRECTION('ref_axis',(0.,0.,1.));
#14978=DIRECTION('',(-1.,0.,2.16840434497101E-16));
#14979=DIRECTION('center_axis',(0.,1.,0.));
#14980=DIRECTION('ref_axis',(0.,0.,1.));
#14981=DIRECTION('',(1.,0.,-2.16840434497101E-16));
#14982=DIRECTION('center_axis',(0.,1.,0.));
#14983=DIRECTION('ref_axis',(0.,0.,1.));
#14984=DIRECTION('center_axis',(0.,-1.,0.));
#14985=DIRECTION('ref_axis',(0.,0.,1.));
#14986=DIRECTION('center_axis',(0.,1.,0.));
#14987=DIRECTION('ref_axis',(0.,0.,1.));
#14988=DIRECTION('',(1.,0.,0.));
#14989=DIRECTION('center_axis',(0.,-1.,0.));
#14990=DIRECTION('ref_axis',(0.,0.,1.));
#14991=DIRECTION('center_axis',(0.,1.,0.));
#14992=DIRECTION('ref_axis',(0.,0.,1.));
#14993=DIRECTION('',(-1.,0.,0.));
#14994=DIRECTION('',(-1.,0.,2.16840434497101E-16));
#14995=DIRECTION('center_axis',(0.,1.,0.));
#14996=DIRECTION('ref_axis',(0.,0.,1.));
#14997=DIRECTION('',(1.,0.,-2.16840434497101E-16));
#14998=DIRECTION('center_axis',(0.,1.,0.));
#14999=DIRECTION('ref_axis',(0.,0.,1.));
#15000=DIRECTION('center_axis',(0.,1.,0.));
#15001=DIRECTION('ref_axis',(0.,0.,1.));
#15002=DIRECTION('',(0.,1.,0.));
#15003=DIRECTION('',(0.,1.,0.));
#15004=DIRECTION('center_axis',(-2.16840434497101E-16,0.,-1.));
#15005=DIRECTION('ref_axis',(-1.,0.,2.16840434497101E-16));
#15006=DIRECTION('',(0.,1.,0.));
#15007=DIRECTION('center_axis',(0.,1.,0.));
#15008=DIRECTION('ref_axis',(0.,0.,1.));
#15009=DIRECTION('',(0.,1.,0.));
#15010=DIRECTION('center_axis',(2.16840434497101E-16,0.,1.));
#15011=DIRECTION('ref_axis',(1.,0.,-2.16840434497101E-16));
#15012=DIRECTION('center_axis',(0.,-1.,0.));
#15013=DIRECTION('ref_axis',(0.,0.,-1.));
#15014=DIRECTION('center_axis',(0.,1.,0.));
#15015=DIRECTION('ref_axis',(0.,0.,1.));
#15016=DIRECTION('center_axis',(1.,0.,0.));
#15017=DIRECTION('ref_axis',(0.,0.,-1.));
#15018=DIRECTION('center_axis',(-1.,0.,0.));
#15019=DIRECTION('ref_axis',(0.,0.,1.));
#15020=DIRECTION('center_axis',(1.,0.,0.));
#15021=DIRECTION('ref_axis',(0.,0.,-1.));
#15022=DIRECTION('center_axis',(-1.,0.,0.));
#15023=DIRECTION('ref_axis',(0.,0.,1.));
#15024=DIRECTION('center_axis',(0.,1.,0.));
#15025=DIRECTION('ref_axis',(0.,0.,1.));
#15026=DIRECTION('center_axis',(0.,-1.,0.));
#15027=DIRECTION('ref_axis',(0.,0.,1.));
#15028=DIRECTION('center_axis',(0.,1.,0.));
#15029=DIRECTION('ref_axis',(0.,0.,1.));
#15030=DIRECTION('',(0.,0.,1.));
#15031=DIRECTION('center_axis',(0.,1.,0.));
#15032=DIRECTION('ref_axis',(0.,0.,1.));
#15033=DIRECTION('',(0.,0.,1.));
#15034=DIRECTION('center_axis',(0.,-1.,0.));
#15035=DIRECTION('ref_axis',(0.,0.,1.));
#15036=DIRECTION('center_axis',(0.,1.,0.));
#15037=DIRECTION('ref_axis',(0.,0.,1.));
#15038=DIRECTION('center_axis',(-1.,0.,0.));
#15039=DIRECTION('ref_axis',(0.,0.,1.));
#15040=DIRECTION('',(0.,-1.,0.));
#15041=DIRECTION('center_axis',(0.,-1.,0.));
#15042=DIRECTION('ref_axis',(0.,0.,-1.));
#15043=DIRECTION('center_axis',(0.,-1.,0.));
#15044=DIRECTION('ref_axis',(0.,0.,-1.));
#15045=DIRECTION('center_axis',(0.,1.,0.));
#15046=DIRECTION('ref_axis',(0.,0.,-1.));
#15047=DIRECTION('',(0.,0.,1.));
#15048=DIRECTION('center_axis',(0.,-1.,0.));
#15049=DIRECTION('ref_axis',(0.,0.,-1.));
#15050=DIRECTION('',(0.,0.,1.));
#15051=DIRECTION('center_axis',(0.,-1.,0.));
#15052=DIRECTION('ref_axis',(0.,0.,-1.));
#15053=DIRECTION('center_axis',(0.,1.,0.));
#15054=DIRECTION('ref_axis',(0.,0.,-1.));
#15055=DIRECTION('center_axis',(1.,0.,0.));
#15056=DIRECTION('ref_axis',(0.,0.,-1.));
#15057=DIRECTION('',(0.,-1.,0.));
#15058=DIRECTION('center_axis',(0.,-1.,0.));
#15059=DIRECTION('ref_axis',(0.,0.,-1.));
#15060=DIRECTION('center_axis',(0.,-1.,0.));
#15061=DIRECTION('ref_axis',(0.,0.,-1.));
#15062=DIRECTION('center_axis',(0.,-1.,0.));
#15063=DIRECTION('ref_axis',(0.,0.,-1.));
#15064=DIRECTION('center_axis',(0.,1.,0.));
#15065=DIRECTION('ref_axis',(0.,0.,1.));
#15066=DIRECTION('center_axis',(0.,1.,0.));
#15067=DIRECTION('ref_axis',(0.,0.,1.));
#15068=DIRECTION('center_axis',(0.,1.,0.));
#15069=DIRECTION('ref_axis',(0.,0.,1.));
#18178=CARTESIAN_POINT('',(0.,0.,0.));
#18179=CARTESIAN_POINT('Origin',(10.,0.,16.));
#18180=CARTESIAN_POINT('',(-6.,-2.75545529808154E-16,13.75));
#18181=CARTESIAN_POINT('Origin',(-6.00000000000001,0.,16.));
#18182=CARTESIAN_POINT('',(-12.,-2.75545529808154E-16,13.75));
#18183=CARTESIAN_POINT('',(10.,-2.75545529808154E-16,13.75));
#18184=CARTESIAN_POINT('Origin',(-12.,0.,16.));
#18185=CARTESIAN_POINT('Origin',(10.,-3.91886975727153E-15,-16.));
#18186=CARTESIAN_POINT('',(12.,-4.19441528707969E-15,-18.25));
#18187=CARTESIAN_POINT('Origin',(12.,-3.91886975727153E-15,-16.));
#18188=CARTESIAN_POINT('',(6.,-4.19441528707969E-15,-18.25));
#18189=CARTESIAN_POINT('',(10.,-4.19441528707969E-15,-18.25));
#18190=CARTESIAN_POINT('Origin',(6.,-3.91886975727153E-15,-16.));
#18191=CARTESIAN_POINT('Origin',(10.,13.,0.));
#18192=CARTESIAN_POINT('',(10.,13.,8.));
#18193=CARTESIAN_POINT('',(10.,13.,-17.));
#18194=CARTESIAN_POINT('',(10.,13.,0.));
#18195=CARTESIAN_POINT('',(10.,3.95,8.));
#18196=CARTESIAN_POINT('',(10.,3.95,8.));
#18197=CARTESIAN_POINT('',(10.,3.95,-22.));
#18198=CARTESIAN_POINT('',(10.,3.95,0.));
#18199=CARTESIAN_POINT('',(10.,8.,-22.));
#18200=CARTESIAN_POINT('',(10.,13.,-22.));
#18201=CARTESIAN_POINT('Origin',(10.,8.,-17.));
#18202=CARTESIAN_POINT('Origin',(-10.,13.,0.));
#18203=CARTESIAN_POINT('',(-10.,13.,17.));
#18204=CARTESIAN_POINT('',(-10.,13.,-8.));
#18205=CARTESIAN_POINT('',(-10.,13.,0.));
#18206=CARTESIAN_POINT('',(-10.,3.95,-8.));
#18207=CARTESIAN_POINT('',(-10.,3.95,-8.));
#18208=CARTESIAN_POINT('',(-10.,3.95,22.));
#18209=CARTESIAN_POINT('',(-10.,3.95,0.));
#18210=CARTESIAN_POINT('',(-10.,8.,22.));
#18211=CARTESIAN_POINT('',(-10.,13.,22.));
#18212=CARTESIAN_POINT('Origin',(-10.,8.,17.));
#18213=CARTESIAN_POINT('Origin',(-10.,13.,0.));
#18214=CARTESIAN_POINT('',(-10.,-3.95,-8.));
#18215=CARTESIAN_POINT('',(-10.,-3.95,22.));
#18216=CARTESIAN_POINT('',(-10.,-3.95,0.));
#18217=CARTESIAN_POINT('',(-10.,-13.,-8.));
#18218=CARTESIAN_POINT('',(-10.,-13.,-8.));
#18219=CARTESIAN_POINT('',(-10.,-13.,17.));
#18220=CARTESIAN_POINT('',(-10.,-13.,0.));
#18221=CARTESIAN_POINT('',(-10.,-7.99999999999999,22.));
#18222=CARTESIAN_POINT('Origin',(-10.,-8.,17.));
#18223=CARTESIAN_POINT('',(-10.,13.,22.));
#18224=CARTESIAN_POINT('Origin',(0.,13.,22.));
#18225=CARTESIAN_POINT('',(-12.,3.95,22.));
#18226=CARTESIAN_POINT('',(-12.,3.95,22.));
#18227=CARTESIAN_POINT('',(-12.,-3.95,22.));
#18228=CARTESIAN_POINT('',(-12.,0.,22.));
#18229=CARTESIAN_POINT('',(-12.,-3.95,22.));
#18230=CARTESIAN_POINT('',(-6.00000000000001,-7.99999999999999,22.));
#18231=CARTESIAN_POINT('',(0.,-8.,22.));
#18232=CARTESIAN_POINT('',(-6.00000000000001,8.,22.));
#18233=CARTESIAN_POINT('',(-6.00000000000001,13.,22.));
#18234=CARTESIAN_POINT('',(-10.,8.,22.));
#18235=CARTESIAN_POINT('Origin',(-6.,13.,-2.60208521396521E-15));
#18236=CARTESIAN_POINT('',(-6.00000000000001,-13.,17.));
#18237=CARTESIAN_POINT('Origin',(-6.00000000000001,-8.,17.));
#18238=CARTESIAN_POINT('',(-6.,-13.,12.));
#18239=CARTESIAN_POINT('',(-6.,-13.,-2.60208521396521E-15));
#18240=CARTESIAN_POINT('',(-6.,13.,12.));
#18241=CARTESIAN_POINT('',(-6.,13.,12.));
#18242=CARTESIAN_POINT('',(-6.00000000000001,13.,17.));
#18243=CARTESIAN_POINT('',(-6.,13.,-2.60208521396521E-15));
#18244=CARTESIAN_POINT('Origin',(-6.00000000000001,8.,17.));
#18245=CARTESIAN_POINT('Origin',(1.73472347597681E-15,13.,10.));
#18246=CARTESIAN_POINT('',(8.,-13.,10.));
#18247=CARTESIAN_POINT('',(-4.,-13.,10.));
#18248=CARTESIAN_POINT('',(1.73472347597681E-15,-13.,10.));
#18249=CARTESIAN_POINT('',(8.,-3.95,10.));
#18250=CARTESIAN_POINT('',(8.,-3.95,10.));
#18251=CARTESIAN_POINT('',(10.,-3.95,10.));
#18252=CARTESIAN_POINT('',(12.,-3.95,10.));
#18253=CARTESIAN_POINT('',(10.,3.95,10.));
#18254=CARTESIAN_POINT('',(10.,13.,10.));
#18255=CARTESIAN_POINT('',(8.,3.95,10.));
#18256=CARTESIAN_POINT('',(12.,3.95,10.));
#18257=CARTESIAN_POINT('',(8.,13.,10.));
#18258=CARTESIAN_POINT('',(8.,13.,10.));
#18259=CARTESIAN_POINT('',(-4.,13.,10.));
#18260=CARTESIAN_POINT('',(1.73472347597681E-15,13.,10.));
#18261=CARTESIAN_POINT('',(-4.,-13.,10.));
#18262=CARTESIAN_POINT('Origin',(10.,13.,0.));
#18263=CARTESIAN_POINT('',(10.,-3.94999999999999,-22.));
#18264=CARTESIAN_POINT('',(10.,-3.95,8.));
#18265=CARTESIAN_POINT('',(10.,-3.95,0.));
#18266=CARTESIAN_POINT('',(10.,-13.,8.));
#18267=CARTESIAN_POINT('',(10.,-13.,8.));
#18268=CARTESIAN_POINT('',(10.,-13.,-17.));
#18269=CARTESIAN_POINT('',(10.,-13.,0.));
#18270=CARTESIAN_POINT('',(10.,-7.99999999999999,-22.));
#18271=CARTESIAN_POINT('Origin',(10.,-8.,-17.));
#18272=CARTESIAN_POINT('',(10.,13.,-22.));
#18273=CARTESIAN_POINT('Origin',(0.,13.,-22.));
#18274=CARTESIAN_POINT('',(6.,8.,-22.));
#18275=CARTESIAN_POINT('',(6.,-7.99999999999999,-22.));
#18276=CARTESIAN_POINT('',(6.,13.,-22.));
#18277=CARTESIAN_POINT('',(10.,8.,-22.));
#18278=CARTESIAN_POINT('',(12.,3.95,-22.));
#18279=CARTESIAN_POINT('',(12.,3.95,-22.));
#18280=CARTESIAN_POINT('',(12.,-3.95,-22.));
#18281=CARTESIAN_POINT('',(12.,0.,-22.));
#18282=CARTESIAN_POINT('',(12.,-3.95,-22.));
#18283=CARTESIAN_POINT('',(0.,-8.,-22.));
#18284=CARTESIAN_POINT('Origin',(6.,13.,0.));
#18285=CARTESIAN_POINT('',(6.,13.,-12.));
#18286=CARTESIAN_POINT('',(6.,13.,-17.));
#18287=CARTESIAN_POINT('',(6.,13.,0.));
#18288=CARTESIAN_POINT('Origin',(6.,8.,-17.));
#18289=CARTESIAN_POINT('',(6.,-13.,-17.));
#18290=CARTESIAN_POINT('Origin',(6.,-8.,-17.));
#18291=CARTESIAN_POINT('',(6.,-13.,-12.));
#18292=CARTESIAN_POINT('',(6.,-13.,0.));
#18293=CARTESIAN_POINT('',(6.,13.,-12.));
#18294=CARTESIAN_POINT('Origin',(0.,13.,-10.));
#18295=CARTESIAN_POINT('',(4.,-13.,-10.));
#18296=CARTESIAN_POINT('',(-8.,-13.,-10.));
#18297=CARTESIAN_POINT('',(0.,-13.,-10.));
#18298=CARTESIAN_POINT('',(-8.,-3.95,-10.));
#18299=CARTESIAN_POINT('',(-8.,-3.95,-10.));
#18300=CARTESIAN_POINT('',(-10.,-3.95,-10.));
#18301=CARTESIAN_POINT('',(-12.,-3.95,-10.));
#18302=CARTESIAN_POINT('',(-10.,3.95,-10.));
#18303=CARTESIAN_POINT('',(-10.,3.95,-10.));
#18304=CARTESIAN_POINT('',(-8.,3.95,-10.));
#18305=CARTESIAN_POINT('',(-12.,3.95,-10.));
#18306=CARTESIAN_POINT('',(-8.,13.,-10.));
#18307=CARTESIAN_POINT('',(-8.,13.,-10.));
#18308=CARTESIAN_POINT('',(4.,13.,-10.));
#18309=CARTESIAN_POINT('',(0.,13.,-10.));
#18310=CARTESIAN_POINT('',(4.,13.,-10.));
#18311=CARTESIAN_POINT('Origin',(0.,13.,0.));
#18312=CARTESIAN_POINT('Origin',(-8.,13.,-8.));
#18313=CARTESIAN_POINT('',(-6.00000000000001,13.,17.));
#18314=CARTESIAN_POINT('Origin',(-4.,13.,12.));
#18315=CARTESIAN_POINT('Origin',(8.,13.,8.));
#18316=CARTESIAN_POINT('',(6.,13.,-17.));
#18317=CARTESIAN_POINT('Origin',(4.,13.,-12.));
#18318=CARTESIAN_POINT('',(-4.,13.,-4.));
#18319=CARTESIAN_POINT('',(-4.,13.,4.));
#18320=CARTESIAN_POINT('Origin',(-4.,13.,0.));
#18321=CARTESIAN_POINT('',(4.,13.,-4.));
#18322=CARTESIAN_POINT('',(-4.,13.,-4.));
#18323=CARTESIAN_POINT('',(4.,13.,4.));
#18324=CARTESIAN_POINT('Origin',(4.,13.,-1.46957615897682E-15));
#18325=CARTESIAN_POINT('',(-4.,13.,4.));
#18326=CARTESIAN_POINT('Origin',(0.,-13.,0.));
#18327=CARTESIAN_POINT('Origin',(-8.,-13.,-8.));
#18328=CARTESIAN_POINT('Origin',(4.,-13.,-12.));
#18329=CARTESIAN_POINT('',(0.,-13.,-17.));
#18330=CARTESIAN_POINT('Origin',(8.,-13.,8.));
#18331=CARTESIAN_POINT('Origin',(-4.,-13.,12.));
#18332=CARTESIAN_POINT('',(0.,-13.,17.));
#18333=CARTESIAN_POINT('',(4.,-13.,-4.));
#18334=CARTESIAN_POINT('',(-4.,-13.,-4.));
#18335=CARTESIAN_POINT('',(-4.,-13.,-4.));
#18336=CARTESIAN_POINT('',(-4.,-13.,4.));
#18337=CARTESIAN_POINT('Origin',(-4.,-13.,0.));
#18338=CARTESIAN_POINT('',(4.,-13.,4.));
#18339=CARTESIAN_POINT('',(-4.,-13.,4.));
#18340=CARTESIAN_POINT('Origin',(4.,-13.,-1.46957615897682E-15));
#18341=CARTESIAN_POINT('Origin',(-4.,-13.,0.));
#18342=CARTESIAN_POINT('',(-4.,-13.,4.));
#18343=CARTESIAN_POINT('',(-4.,-13.,-4.));
#18344=CARTESIAN_POINT('Origin',(-4.,-13.,-4.));
#18345=CARTESIAN_POINT('',(4.,-13.,-4.));
#18346=CARTESIAN_POINT('Origin',(4.,-13.,-1.46957615897682E-15));
#18347=CARTESIAN_POINT('',(4.,-13.,4.));
#18348=CARTESIAN_POINT('Origin',(-4.,-13.,4.));
#18349=CARTESIAN_POINT('Origin',(4.,13.,-12.));
#18350=CARTESIAN_POINT('Origin',(-4.,13.,12.));
#18351=CARTESIAN_POINT('Origin',(0.,8.,-17.));
#18352=CARTESIAN_POINT('Origin',(0.,-8.,-17.));
#18353=CARTESIAN_POINT('Origin',(0.,-8.,17.));
#18354=CARTESIAN_POINT('Origin',(0.,8.,17.));
#18355=CARTESIAN_POINT('Origin',(-12.,3.95,0.));
#18356=CARTESIAN_POINT('Origin',(-8.,3.95,-8.));
#18357=CARTESIAN_POINT('',(-12.,3.95,-8.));
#18358=CARTESIAN_POINT('Origin',(-10.,3.95,-8.));
#18359=CARTESIAN_POINT('',(-12.,3.95,0.));
#18360=CARTESIAN_POINT('Origin',(-12.,-3.95,0.));
#18361=CARTESIAN_POINT('',(-12.,-3.95,-8.));
#18362=CARTESIAN_POINT('',(-12.,-3.95,0.));
#18363=CARTESIAN_POINT('Origin',(-10.,-3.95,-8.));
#18364=CARTESIAN_POINT('Origin',(-8.,-3.95,-8.));
#18365=CARTESIAN_POINT('Origin',(-12.,0.,0.));
#18366=CARTESIAN_POINT('',(-12.,-3.95,-8.));
#18367=CARTESIAN_POINT('Origin',(12.,3.95,0.));
#18368=CARTESIAN_POINT('Origin',(8.,3.95,8.));
#18369=CARTESIAN_POINT('',(12.,3.95,8.));
#18370=CARTESIAN_POINT('Origin',(10.,3.95,8.));
#18371=CARTESIAN_POINT('',(12.,3.95,0.));
#18372=CARTESIAN_POINT('Origin',(12.,-3.95,0.));
#18373=CARTESIAN_POINT('',(12.,-3.95,8.));
#18374=CARTESIAN_POINT('',(12.,-3.95,0.));
#18375=CARTESIAN_POINT('Origin',(10.,-3.95,8.));
#18376=CARTESIAN_POINT('Origin',(8.,-3.95,8.));
#18377=CARTESIAN_POINT('Origin',(12.,0.,0.));
#18378=CARTESIAN_POINT('',(12.,0.,8.));
#18379=CARTESIAN_POINT('Origin',(-8.,13.,-8.));
#18380=CARTESIAN_POINT('Origin',(-10.,13.,-8.));
#18381=CARTESIAN_POINT('Origin',(-8.,13.,-8.));
#18382=CARTESIAN_POINT('Origin',(8.,13.,8.));
#18383=CARTESIAN_POINT('Origin',(10.,13.,8.));
#18384=CARTESIAN_POINT('Origin',(8.,13.,8.));
#18844=UNCERTAINTY_MEASURE_WITH_UNIT(LENGTH_MEASURE(0.01),#18868,
'DISTANCE_ACCURACY_VALUE',
'Maximum model space distance between geometric entities at asserted c
onnectivities');
#18849=UNCERTAINTY_MEASURE_WITH_UNIT(LENGTH_MEASURE(0.01),#18868,
'DISTANCE_ACCURACY_VALUE',
'Maximum model space distance between geometric entities at asserted c
onnectivities');
#18862=(
GEOMETRIC_REPRESENTATION_CONTEXT(3)
GLOBAL_UNCERTAINTY_ASSIGNED_CONTEXT((#18844))
GLOBAL_UNIT_ASSIGNED_CONTEXT((#18868,#18870,#18871))
REPRESENTATION_CONTEXT('','3D')
);
#18867=(
GEOMETRIC_REPRESENTATION_CONTEXT(3)
GLOBAL_UNCERTAINTY_ASSIGNED_CONTEXT((#18849))
GLOBAL_UNIT_ASSIGNED_CONTEXT((#18868,#18870,#18871))
REPRESENTATION_CONTEXT('','3D')
);
#18868=(
LENGTH_UNIT()
NAMED_UNIT(*)
SI_UNIT(.MILLI.,.METRE.)
);
#18870=(
NAMED_UNIT(*)
PLANE_ANGLE_UNIT()
SI_UNIT($,.RADIAN.)
);
#18871=(
NAMED_UNIT(*)
SI_UNIT($,.STERADIAN.)
SOLID_ANGLE_UNIT()
);
#18884=SHAPE_DEFINITION_REPRESENTATION(#18901,#18946);
#18901=PRODUCT_DEFINITION_SHAPE('',$,#18964);
#18946=SHAPE_REPRESENTATION('',(#12015),#18862);
#18951=PRODUCT_DEFINITION_CONTEXT('part definition',#19004,'design');
#18964=PRODUCT_DEFINITION('Arm Clamp Block','Arm Clamp Block',#18981,#18951);
#18981=PRODUCT_DEFINITION_FORMATION('',$,#19018);
#19004=APPLICATION_CONTEXT(
'Core Data for Automotive Mechanical Design Process');
#19005=PRODUCT_CONTEXT('part definition',#19004,'mechanical');
#19018=PRODUCT('Arm Clamp Block','Arm Clamp Block',$,(#19005));
#19026=PRESENTATION_STYLE_ASSIGNMENT((#19032));
#19032=SURFACE_STYLE_USAGE(.BOTH.,#19038);
#19038=SURFACE_SIDE_STYLE('',(#19044));
#19044=SURFACE_STYLE_FILL_AREA(#19050);
#19050=FILL_AREA_STYLE('Opaque(227,224,212)',(#19056));
#19056=FILL_AREA_STYLE_COLOUR('Opaque(227,224,212)',#19062);
#19062=COLOUR_RGB('Opaque(227,224,212)',0.890196078431372,0.87843137254902,
0.831372549019608);
ENDSEC;
END-ISO-10303-21;
